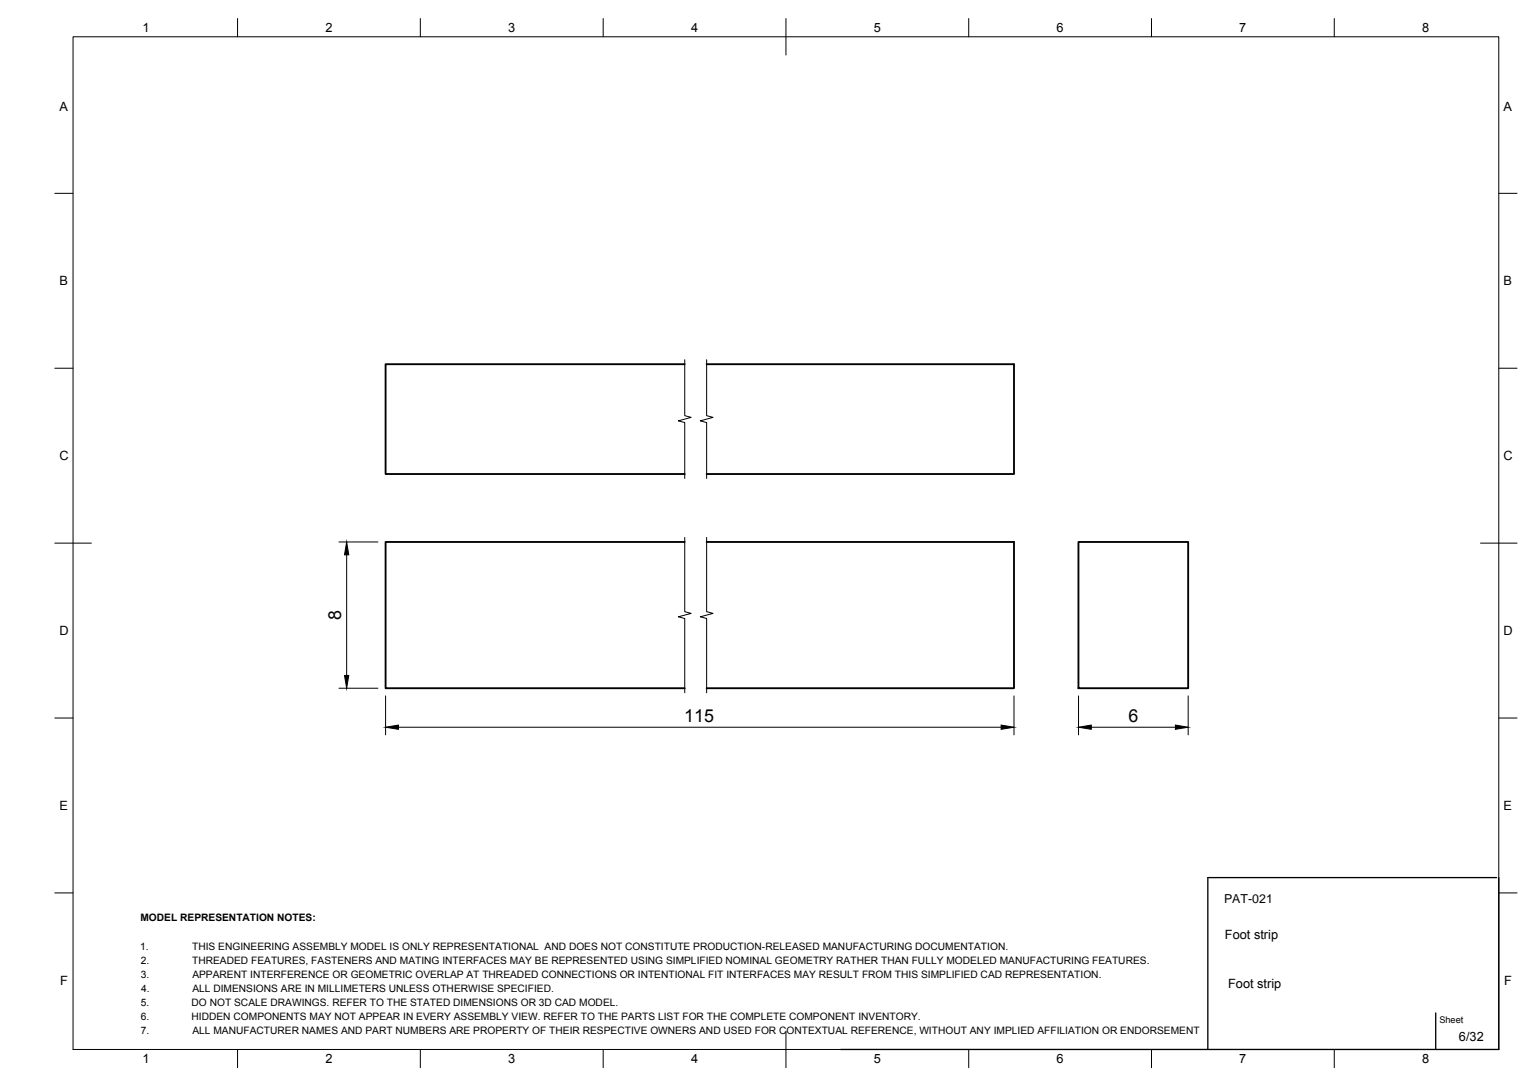
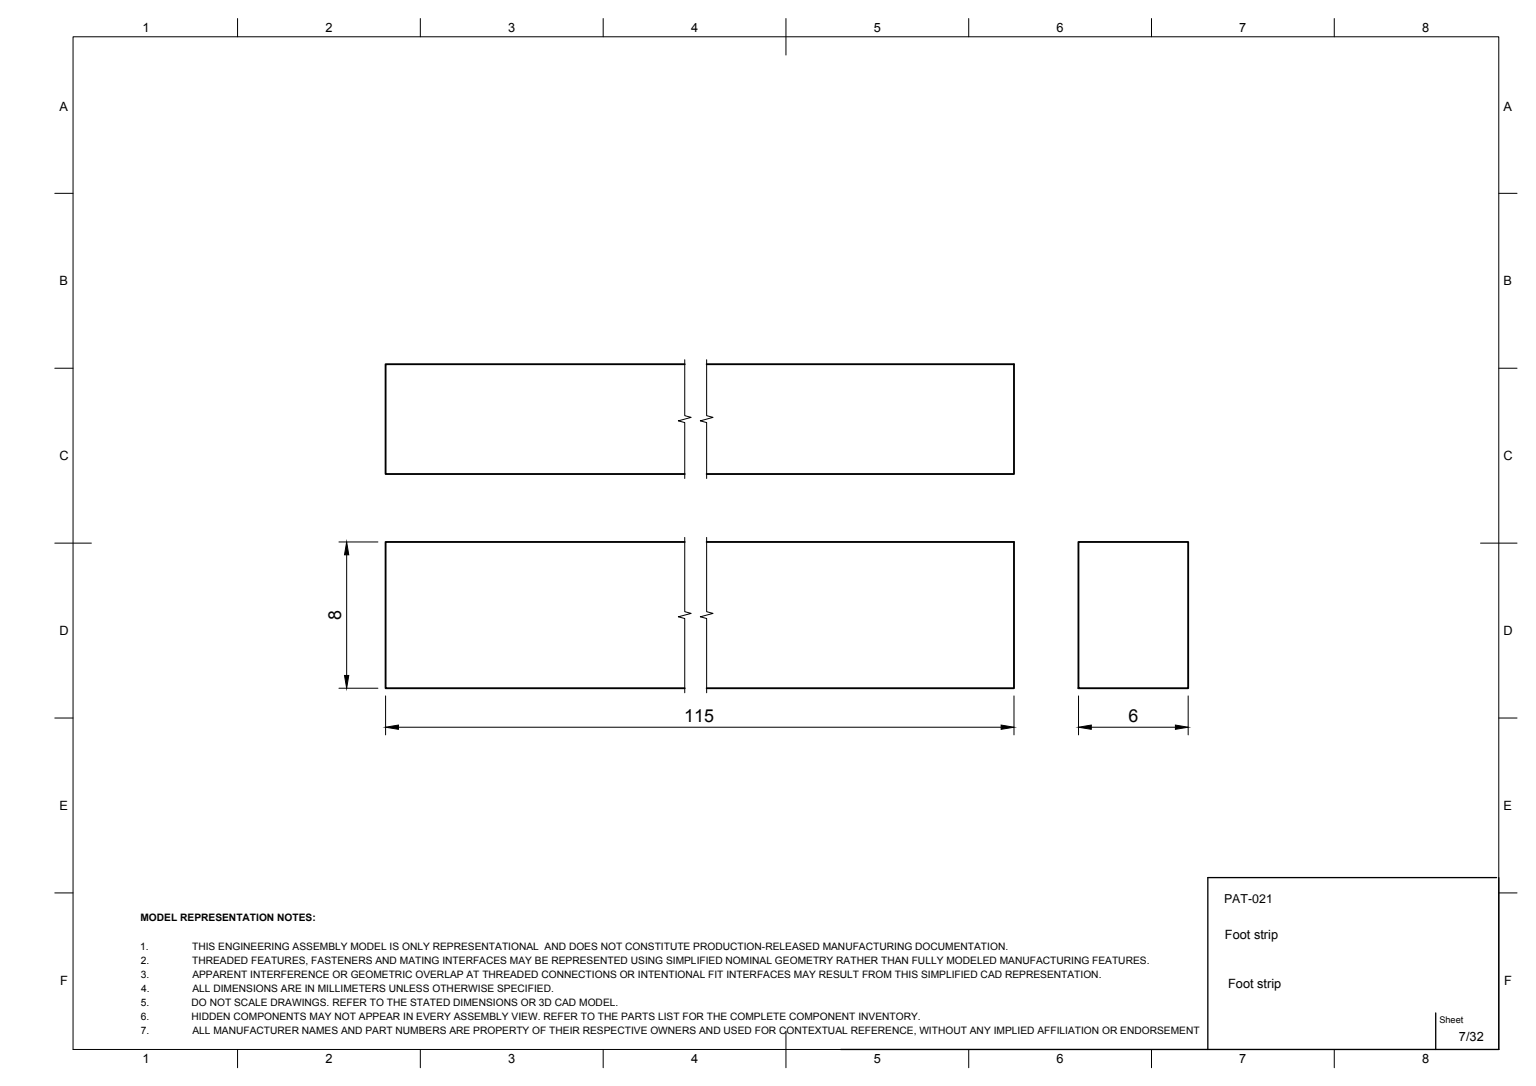
ISO-10303-21;
HEADER;
/* Generated by software containing ST-Developer
 * from STEP Tools, Inc. (www.steptools.com) 
 */

FILE_DESCRIPTION(
/* description */ ('Chain-less indexing wheel (Geneva) drive'),
/* implementation_level */ '2;1');

FILE_NAME(
/* name */ 'Foot strip.step',
/* time_stamp */ '2026-10-28T03:25:22-07:00',
/* author */ (''),
/* organization */ (''),
/* preprocessor_version */ 'ST-DEVELOPER v20.2',
/* originating_system */ 'Autodesk Translation Framework v15.17.0.0',
/* authorisation */ '');

FILE_SCHEMA (('AUTOMOTIVE_DESIGN { 1 0 10303 214 3 1 1 }'));
ENDSEC;

DATA;
#10=MECHANICAL_DESIGN_GEOMETRIC_PRESENTATION_REPRESENTATION('',(#304),#10957);
#254=SHAPE_REPRESENTATION_RELATIONSHIP('SRR','None',#11067,#279);
#279=ADVANCED_BREP_SHAPE_REPRESENTATION('',(#337),#10930);
#304=STYLED_ITEM('',(#11273),#337);
#337=MANIFOLD_SOLID_BREP('Body1',#5700);
#478=PLANE('',#6032);
#479=PLANE('',#6033);
#480=PLANE('',#6034);
#481=PLANE('',#6035);
#482=PLANE('',#6036);
#483=PLANE('',#6037);
#662=FACE_OUTER_BOUND('',#1003,.T.);
#663=FACE_OUTER_BOUND('',#1004,.T.);
#664=FACE_OUTER_BOUND('',#1005,.T.);
#665=FACE_OUTER_BOUND('',#1006,.T.);
#666=FACE_OUTER_BOUND('',#1007,.T.);
#667=FACE_OUTER_BOUND('',#1008,.T.);
#1003=EDGE_LOOP('',(#3795,#3796,#3797,#3798));
#1004=EDGE_LOOP('',(#3799,#3800,#3801,#3802));
#1005=EDGE_LOOP('',(#3803,#3804,#3805,#3806));
#1006=EDGE_LOOP('',(#3807,#3808,#3809,#3810));
#1007=EDGE_LOOP('',(#3811,#3812,#3813,#3814));
#1008=EDGE_LOOP('',(#3815,#3816,#3817,#3818));
#1439=LINE('',#8658,#1813);
#1440=LINE('',#8660,#1814);
#1441=LINE('',#8662,#1815);
#1442=LINE('',#8663,#1816);
#1443=LINE('',#8666,#1817);
#1444=LINE('',#8668,#1818);
#1445=LINE('',#8669,#1819);
#1446=LINE('',#8672,#1820);
#1447=LINE('',#8674,#1821);
#1448=LINE('',#8675,#1822);
#1449=LINE('',#8677,#1823);
#1450=LINE('',#8678,#1824);
#1813=VECTOR('',#6811,1.);
#1814=VECTOR('',#6812,1.);
#1815=VECTOR('',#6813,1.);
#1816=VECTOR('',#6814,1.);
#1817=VECTOR('',#6817,1.);
#1818=VECTOR('',#6818,1.);
#1819=VECTOR('',#6819,1.);
#1820=VECTOR('',#6822,1.);
#1821=VECTOR('',#6823,1.);
#1822=VECTOR('',#6824,1.);
#1823=VECTOR('',#6827,1.);
#1824=VECTOR('',#6828,1.);
#2521=VERTEX_POINT('',#8656);
#2522=VERTEX_POINT('',#8657);
#2523=VERTEX_POINT('',#8659);
#2524=VERTEX_POINT('',#8661);
#2525=VERTEX_POINT('',#8665);
#2526=VERTEX_POINT('',#8667);
#2527=VERTEX_POINT('',#8671);
#2528=VERTEX_POINT('',#8673);
#3023=EDGE_CURVE('',#2521,#2522,#1439,.T.);
#3024=EDGE_CURVE('',#2522,#2523,#1440,.T.);
#3025=EDGE_CURVE('',#2524,#2523,#1441,.T.);
#3026=EDGE_CURVE('',#2521,#2524,#1442,.T.);
#3027=EDGE_CURVE('',#2525,#2521,#1443,.T.);
#3028=EDGE_CURVE('',#2526,#2524,#1444,.T.);
#3029=EDGE_CURVE('',#2525,#2526,#1445,.T.);
#3030=EDGE_CURVE('',#2527,#2525,#1446,.T.);
#3031=EDGE_CURVE('',#2528,#2526,#1447,.T.);
#3032=EDGE_CURVE('',#2527,#2528,#1448,.T.);
#3033=EDGE_CURVE('',#2522,#2527,#1449,.T.);
#3034=EDGE_CURVE('',#2523,#2528,#1450,.T.);
#3795=ORIENTED_EDGE('',*,*,#3023,.T.);
#3796=ORIENTED_EDGE('',*,*,#3024,.T.);
#3797=ORIENTED_EDGE('',*,*,#3025,.F.);
#3798=ORIENTED_EDGE('',*,*,#3026,.F.);
#3799=ORIENTED_EDGE('',*,*,#3027,.T.);
#3800=ORIENTED_EDGE('',*,*,#3026,.T.);
#3801=ORIENTED_EDGE('',*,*,#3028,.F.);
#3802=ORIENTED_EDGE('',*,*,#3029,.F.);
#3803=ORIENTED_EDGE('',*,*,#3030,.T.);
#3804=ORIENTED_EDGE('',*,*,#3029,.T.);
#3805=ORIENTED_EDGE('',*,*,#3031,.F.);
#3806=ORIENTED_EDGE('',*,*,#3032,.F.);
#3807=ORIENTED_EDGE('',*,*,#3033,.T.);
#3808=ORIENTED_EDGE('',*,*,#3032,.T.);
#3809=ORIENTED_EDGE('',*,*,#3034,.F.);
#3810=ORIENTED_EDGE('',*,*,#3024,.F.);
#3811=ORIENTED_EDGE('',*,*,#3034,.T.);
#3812=ORIENTED_EDGE('',*,*,#3031,.T.);
#3813=ORIENTED_EDGE('',*,*,#3028,.T.);
#3814=ORIENTED_EDGE('',*,*,#3025,.T.);
#3815=ORIENTED_EDGE('',*,*,#3033,.F.);
#3816=ORIENTED_EDGE('',*,*,#3023,.F.);
#3817=ORIENTED_EDGE('',*,*,#3027,.F.);
#3818=ORIENTED_EDGE('',*,*,#3030,.F.);
#5376=ADVANCED_FACE('',(#662),#478,.T.);
#5377=ADVANCED_FACE('',(#663),#479,.T.);
#5378=ADVANCED_FACE('',(#664),#480,.T.);
#5379=ADVANCED_FACE('',(#665),#481,.T.);
#5380=ADVANCED_FACE('',(#666),#482,.T.);
#5381=ADVANCED_FACE('',(#667),#483,.F.);
#5700=CLOSED_SHELL('',(#5376,#5377,#5378,#5379,#5380,#5381));
#6031=AXIS2_PLACEMENT_3D('',#8654,#6807,#6808);
#6032=AXIS2_PLACEMENT_3D('',#8655,#6809,#6810);
#6033=AXIS2_PLACEMENT_3D('',#8664,#6815,#6816);
#6034=AXIS2_PLACEMENT_3D('',#8670,#6820,#6821);
#6035=AXIS2_PLACEMENT_3D('',#8676,#6825,#6826);
#6036=AXIS2_PLACEMENT_3D('',#8679,#6829,#6830);
#6037=AXIS2_PLACEMENT_3D('',#8680,#6831,#6832);
#6807=DIRECTION('axis',(0.,0.,1.));
#6808=DIRECTION('refdir',(1.,0.,0.));
#6809=DIRECTION('center_axis',(0.,1.,0.));
#6810=DIRECTION('ref_axis',(-1.,0.,0.));
#6811=DIRECTION('',(-1.,0.,0.));
#6812=DIRECTION('',(0.,0.,1.));
#6813=DIRECTION('',(-1.,0.,0.));
#6814=DIRECTION('',(0.,0.,1.));
#6815=DIRECTION('center_axis',(1.,0.,0.));
#6816=DIRECTION('ref_axis',(0.,1.,0.));
#6817=DIRECTION('',(0.,1.,0.));
#6818=DIRECTION('',(0.,1.,0.));
#6819=DIRECTION('',(0.,0.,1.));
#6820=DIRECTION('center_axis',(0.,-1.,0.));
#6821=DIRECTION('ref_axis',(1.,0.,0.));
#6822=DIRECTION('',(1.,0.,0.));
#6823=DIRECTION('',(1.,0.,0.));
#6824=DIRECTION('',(0.,0.,1.));
#6825=DIRECTION('center_axis',(-1.,0.,0.));
#6826=DIRECTION('ref_axis',(0.,-1.,0.));
#6827=DIRECTION('',(0.,-1.,0.));
#6828=DIRECTION('',(0.,-1.,0.));
#6829=DIRECTION('center_axis',(0.,0.,1.));
#6830=DIRECTION('ref_axis',(1.,0.,0.));
#6831=DIRECTION('center_axis',(0.,0.,1.));
#6832=DIRECTION('ref_axis',(1.,0.,0.));
#8654=CARTESIAN_POINT('',(0.,0.,0.));
#8655=CARTESIAN_POINT('Origin',(8.,-3.2,-0.6));
#8656=CARTESIAN_POINT('',(8.,-3.2,-0.6));
#8657=CARTESIAN_POINT('',(-3.5,-3.2,-0.6));
#8658=CARTESIAN_POINT('',(8.,-3.2,-0.6));
#8659=CARTESIAN_POINT('',(-3.5,-3.2,0.));
#8660=CARTESIAN_POINT('',(-3.5,-3.2,-0.6));
#8661=CARTESIAN_POINT('',(8.,-3.2,0.));
#8662=CARTESIAN_POINT('',(8.,-3.2,0.));
#8663=CARTESIAN_POINT('',(8.,-3.2,-0.6));
#8664=CARTESIAN_POINT('Origin',(8.,-4.,-0.6));
#8665=CARTESIAN_POINT('',(8.,-4.,-0.6));
#8666=CARTESIAN_POINT('',(8.,-4.,-0.6));
#8667=CARTESIAN_POINT('',(8.,-4.,0.));
#8668=CARTESIAN_POINT('',(8.,-4.,0.));
#8669=CARTESIAN_POINT('',(8.,-4.,-0.6));
#8670=CARTESIAN_POINT('Origin',(-3.5,-4.,-0.6));
#8671=CARTESIAN_POINT('',(-3.5,-4.,-0.6));
#8672=CARTESIAN_POINT('',(-3.5,-4.,-0.6));
#8673=CARTESIAN_POINT('',(-3.5,-4.,0.));
#8674=CARTESIAN_POINT('',(-3.5,-4.,0.));
#8675=CARTESIAN_POINT('',(-3.5,-4.,-0.6));
#8676=CARTESIAN_POINT('Origin',(-3.5,-3.2,-0.6));
#8677=CARTESIAN_POINT('',(-3.5,-3.2,-0.6));
#8678=CARTESIAN_POINT('',(-3.5,-3.2,0.));
#8679=CARTESIAN_POINT('Origin',(2.25,-3.6,0.));
#8680=CARTESIAN_POINT('Origin',(2.25,-3.6,-0.6));
#10899=UNCERTAINTY_MEASURE_WITH_UNIT(LENGTH_MEASURE(0.001),#10958,
'DISTANCE_ACCURACY_VALUE',
'Maximum model space distance between geometric entities at asserted c
onnectivities');
#10926=UNCERTAINTY_MEASURE_WITH_UNIT(LENGTH_MEASURE(0.001),#10958,
'DISTANCE_ACCURACY_VALUE',
'Maximum model space distance between geometric entities at asserted c
onnectivities');
#10930=(
GEOMETRIC_REPRESENTATION_CONTEXT(3)
GLOBAL_UNCERTAINTY_ASSIGNED_CONTEXT((#10899))
GLOBAL_UNIT_ASSIGNED_CONTEXT((#10958,#10960,#10961))
REPRESENTATION_CONTEXT('','3D')
);
#10957=(
GEOMETRIC_REPRESENTATION_CONTEXT(3)
GLOBAL_UNCERTAINTY_ASSIGNED_CONTEXT((#10926))
GLOBAL_UNIT_ASSIGNED_CONTEXT((#10958,#10960,#10961))
REPRESENTATION_CONTEXT('','3D')
);
#10958=(
LENGTH_UNIT()
NAMED_UNIT(*)
SI_UNIT(.CENTI.,.METRE.)
);
#10960=(
NAMED_UNIT(*)
PLANE_ANGLE_UNIT()
SI_UNIT($,.RADIAN.)
);
#10961=(
NAMED_UNIT(*)
SI_UNIT($,.STERADIAN.)
SOLID_ANGLE_UNIT()
);
#10965=SHAPE_DEFINITION_REPRESENTATION(#10995,#11067);
#10995=PRODUCT_DEFINITION_SHAPE('',$,#11098);
#11067=SHAPE_REPRESENTATION('',(#6031),#10930);
#11094=PRODUCT_DEFINITION_CONTEXT('part definition',#11186,'design');
#11098=PRODUCT_DEFINITION('Foot strip','Foot strip',#11128,#11094);
#11128=PRODUCT_DEFINITION_FORMATION('',$,#11191);
#11186=APPLICATION_CONTEXT(
'Core Data for Automotive Mechanical Design Process');
#11187=PRODUCT_CONTEXT('part definition',#11186,'mechanical');
#11191=PRODUCT('Foot strip','Foot strip','Foot strip',(#11187));
#11267=COLOUR_RGB('Light Blue',0.38,0.62,0.78);
#11268=FILL_AREA_STYLE_COLOUR('',#11267);
#11269=FILL_AREA_STYLE('',(#11268));
#11270=SURFACE_STYLE_FILL_AREA(#11269);
#11271=SURFACE_SIDE_STYLE('',(#11270));
#11272=SURFACE_STYLE_USAGE(.BOTH.,#11271);
#11273=PRESENTATION_STYLE_ASSIGNMENT((#11272));
ENDSEC;
END-ISO-10303-21;
